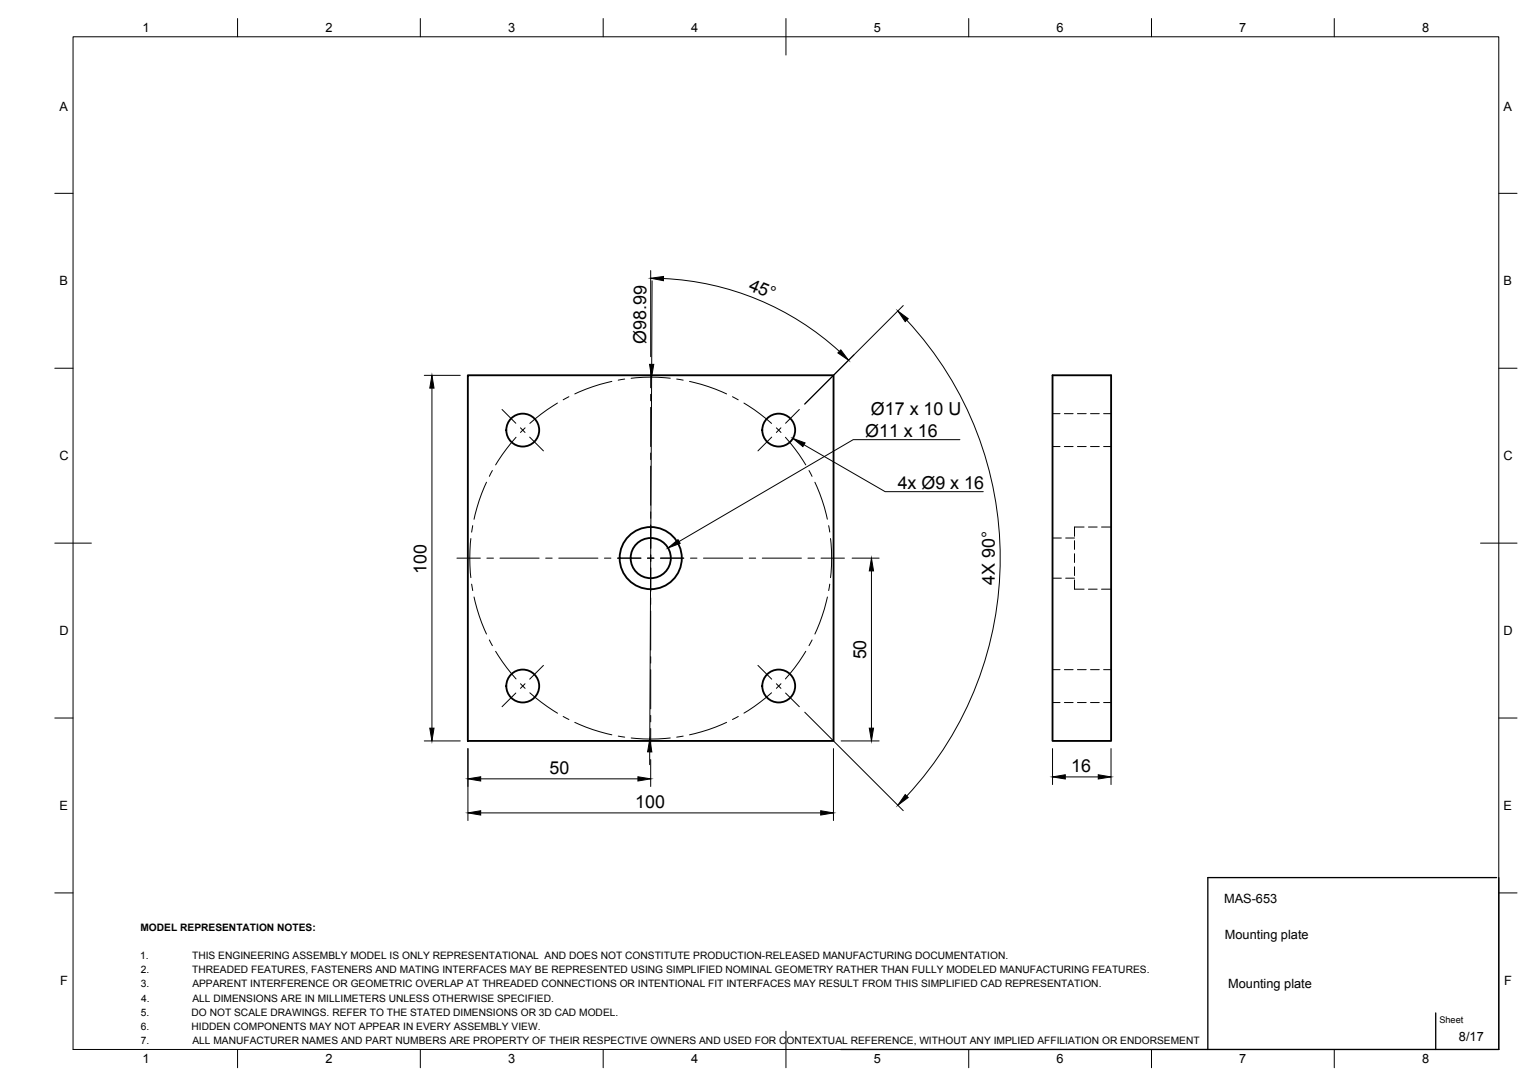
ISO-10303-21;
HEADER;
/* Generated by software containing ST-Developer
 * from STEP Tools, Inc. (www.steptools.com) 
 */

FILE_DESCRIPTION(
/* description */ ('Independent compact industrial fixture table, bolted aluminum worktop
 on connected adjustable support base. Whole-mm nominal dimensions. No
 load rating assigned.'),
/* implementation_level */ '2;1');

FILE_NAME(
/* name */ 'Mounting plate.step',
/* time_stamp */ '2026-11-07T17:47:58-08:00',
/* author */ (''),
/* organization */ (''),
/* preprocessor_version */ 'ST-DEVELOPER v20.2',
/* originating_system */ 'Autodesk Translation Framework v15.17.0.0',
/* authorisation */ '');

FILE_SCHEMA (('AUTOMOTIVE_DESIGN { 1 0 10303 214 3 1 1 }'));
ENDSEC;

DATA;
#10=MECHANICAL_DESIGN_GEOMETRIC_PRESENTATION_REPRESENTATION('',(#2256),#97475);
#2218=SHAPE_REPRESENTATION_RELATIONSHIP('SRR','None',#97612,#2237);
#2237=ADVANCED_BREP_SHAPE_REPRESENTATION('',(#2275),#97462);
#2256=STYLED_ITEM('',(#97722),#2275);
#2275=MANIFOLD_SOLID_BREP('Body1',#21817);
#2328=FACE_BOUND('',#4133,.T.);
#2329=FACE_BOUND('',#4145,.T.);
#2330=FACE_BOUND('',#4146,.T.);
#2331=FACE_BOUND('',#4147,.T.);
#2332=FACE_BOUND('',#4148,.T.);
#2333=FACE_BOUND('',#4149,.T.);
#2334=FACE_BOUND('',#4151,.T.);
#2335=FACE_BOUND('',#4152,.T.);
#2336=FACE_BOUND('',#4153,.T.);
#2337=FACE_BOUND('',#4154,.T.);
#2338=FACE_BOUND('',#4155,.T.);
#2459=PLANE('',#22610);
#2460=PLANE('',#22629);
#2461=PLANE('',#22630);
#2462=PLANE('',#22631);
#2463=PLANE('',#22632);
#2464=PLANE('',#22633);
#2465=PLANE('',#22634);
#2938=FACE_OUTER_BOUND('',#4132,.T.);
#2939=FACE_OUTER_BOUND('',#4134,.T.);
#2940=FACE_OUTER_BOUND('',#4135,.T.);
#2941=FACE_OUTER_BOUND('',#4136,.T.);
#2942=FACE_OUTER_BOUND('',#4137,.T.);
#2943=FACE_OUTER_BOUND('',#4138,.T.);
#2944=FACE_OUTER_BOUND('',#4139,.T.);
#2945=FACE_OUTER_BOUND('',#4140,.T.);
#2946=FACE_OUTER_BOUND('',#4141,.T.);
#2947=FACE_OUTER_BOUND('',#4142,.T.);
#2948=FACE_OUTER_BOUND('',#4143,.T.);
#2949=FACE_OUTER_BOUND('',#4144,.T.);
#2950=FACE_OUTER_BOUND('',#4150,.T.);
#4132=EDGE_LOOP('',(#15422));
#4133=EDGE_LOOP('',(#15423));
#4134=EDGE_LOOP('',(#15424,#15425,#15426,#15427));
#4135=EDGE_LOOP('',(#15428,#15429,#15430,#15431));
#4136=EDGE_LOOP('',(#15432,#15433,#15434,#15435));
#4137=EDGE_LOOP('',(#15436,#15437,#15438,#15439));
#4138=EDGE_LOOP('',(#15440,#15441,#15442,#15443));
#4139=EDGE_LOOP('',(#15444,#15445,#15446,#15447));
#4140=EDGE_LOOP('',(#15448,#15449,#15450,#15451));
#4141=EDGE_LOOP('',(#15452,#15453,#15454,#15455));
#4142=EDGE_LOOP('',(#15456,#15457,#15458,#15459));
#4143=EDGE_LOOP('',(#15460,#15461,#15462,#15463));
#4144=EDGE_LOOP('',(#15464,#15465,#15466,#15467));
#4145=EDGE_LOOP('',(#15468));
#4146=EDGE_LOOP('',(#15469));
#4147=EDGE_LOOP('',(#15470));
#4148=EDGE_LOOP('',(#15471));
#4149=EDGE_LOOP('',(#15472));
#4150=EDGE_LOOP('',(#15473,#15474,#15475,#15476));
#4151=EDGE_LOOP('',(#15477));
#4152=EDGE_LOOP('',(#15478));
#4153=EDGE_LOOP('',(#15479));
#4154=EDGE_LOOP('',(#15480));
#4155=EDGE_LOOP('',(#15481));
#5417=LINE('',#53275,#6631);
#5418=LINE('',#53278,#6632);
#5419=LINE('',#53284,#6633);
#5420=LINE('',#53290,#6634);
#5421=LINE('',#53296,#6635);
#5422=LINE('',#53302,#6636);
#5423=LINE('',#53307,#6637);
#5424=LINE('',#53309,#6638);
#5425=LINE('',#53311,#6639);
#5426=LINE('',#53312,#6640);
#5427=LINE('',#53315,#6641);
#5428=LINE('',#53317,#6642);
#5429=LINE('',#53318,#6643);
#5430=LINE('',#53321,#6644);
#5431=LINE('',#53323,#6645);
#5432=LINE('',#53324,#6646);
#5433=LINE('',#53326,#6647);
#5434=LINE('',#53327,#6648);
#6631=VECTOR('',#25133,8.5);
#6632=VECTOR('',#25136,5.5);
#6633=VECTOR('',#25143,4.5);
#6634=VECTOR('',#25150,4.5);
#6635=VECTOR('',#25157,4.5);
#6636=VECTOR('',#25164,4.5);
#6637=VECTOR('',#25169,10.);
#6638=VECTOR('',#25170,10.);
#6639=VECTOR('',#25171,10.);
#6640=VECTOR('',#25172,10.);
#6641=VECTOR('',#25175,10.);
#6642=VECTOR('',#25176,10.);
#6643=VECTOR('',#25177,10.);
#6644=VECTOR('',#25180,10.);
#6645=VECTOR('',#25181,10.);
#6646=VECTOR('',#25182,10.);
#6647=VECTOR('',#25185,10.);
#6648=VECTOR('',#25186,10.);
#7497=CIRCLE('',#22611,8.5);
#7498=CIRCLE('',#22612,5.5);
#7499=CIRCLE('',#22614,8.5);
#7500=CIRCLE('',#22616,5.5);
#7501=CIRCLE('',#22618,4.5);
#7502=CIRCLE('',#22619,4.5);
#7503=CIRCLE('',#22621,4.5);
#7504=CIRCLE('',#22622,4.5);
#7505=CIRCLE('',#22624,4.5);
#7506=CIRCLE('',#22625,4.5);
#7507=CIRCLE('',#22627,4.5);
#7508=CIRCLE('',#22628,4.5);
#8383=VERTEX_POINT('',#53268);
#8384=VERTEX_POINT('',#53270);
#8385=VERTEX_POINT('',#53273);
#8386=VERTEX_POINT('',#53277);
#8387=VERTEX_POINT('',#53281);
#8388=VERTEX_POINT('',#53283);
#8389=VERTEX_POINT('',#53287);
#8390=VERTEX_POINT('',#53289);
#8391=VERTEX_POINT('',#53293);
#8392=VERTEX_POINT('',#53295);
#8393=VERTEX_POINT('',#53299);
#8394=VERTEX_POINT('',#53301);
#8395=VERTEX_POINT('',#53305);
#8396=VERTEX_POINT('',#53306);
#8397=VERTEX_POINT('',#53308);
#8398=VERTEX_POINT('',#53310);
#8399=VERTEX_POINT('',#53314);
#8400=VERTEX_POINT('',#53316);
#8401=VERTEX_POINT('',#53320);
#8402=VERTEX_POINT('',#53322);
#10968=EDGE_CURVE('',#8383,#8383,#7497,.T.);
#10969=EDGE_CURVE('',#8384,#8384,#7498,.T.);
#10970=EDGE_CURVE('',#8385,#8385,#7499,.T.);
#10971=EDGE_CURVE('',#8385,#8383,#5417,.T.);
#10972=EDGE_CURVE('',#8384,#8386,#5418,.T.);
#10973=EDGE_CURVE('',#8386,#8386,#7500,.T.);
#10974=EDGE_CURVE('',#8387,#8387,#7501,.T.);
#10975=EDGE_CURVE('',#8387,#8388,#5419,.T.);
#10976=EDGE_CURVE('',#8388,#8388,#7502,.T.);
#10977=EDGE_CURVE('',#8389,#8389,#7503,.T.);
#10978=EDGE_CURVE('',#8389,#8390,#5420,.T.);
#10979=EDGE_CURVE('',#8390,#8390,#7504,.T.);
#10980=EDGE_CURVE('',#8391,#8391,#7505,.T.);
#10981=EDGE_CURVE('',#8391,#8392,#5421,.T.);
#10982=EDGE_CURVE('',#8392,#8392,#7506,.T.);
#10983=EDGE_CURVE('',#8393,#8393,#7507,.T.);
#10984=EDGE_CURVE('',#8393,#8394,#5422,.T.);
#10985=EDGE_CURVE('',#8394,#8394,#7508,.T.);
#10986=EDGE_CURVE('',#8395,#8396,#5423,.T.);
#10987=EDGE_CURVE('',#8396,#8397,#5424,.T.);
#10988=EDGE_CURVE('',#8398,#8397,#5425,.T.);
#10989=EDGE_CURVE('',#8395,#8398,#5426,.T.);
#10990=EDGE_CURVE('',#8399,#8395,#5427,.T.);
#10991=EDGE_CURVE('',#8400,#8398,#5428,.T.);
#10992=EDGE_CURVE('',#8399,#8400,#5429,.T.);
#10993=EDGE_CURVE('',#8401,#8399,#5430,.T.);
#10994=EDGE_CURVE('',#8402,#8400,#5431,.T.);
#10995=EDGE_CURVE('',#8401,#8402,#5432,.T.);
#10996=EDGE_CURVE('',#8396,#8401,#5433,.T.);
#10997=EDGE_CURVE('',#8397,#8402,#5434,.T.);
#15422=ORIENTED_EDGE('',*,*,#10968,.F.);
#15423=ORIENTED_EDGE('',*,*,#10969,.T.);
#15424=ORIENTED_EDGE('',*,*,#10970,.F.);
#15425=ORIENTED_EDGE('',*,*,#10971,.T.);
#15426=ORIENTED_EDGE('',*,*,#10968,.T.);
#15427=ORIENTED_EDGE('',*,*,#10971,.F.);
#15428=ORIENTED_EDGE('',*,*,#10969,.F.);
#15429=ORIENTED_EDGE('',*,*,#10972,.T.);
#15430=ORIENTED_EDGE('',*,*,#10973,.F.);
#15431=ORIENTED_EDGE('',*,*,#10972,.F.);
#15432=ORIENTED_EDGE('',*,*,#10974,.F.);
#15433=ORIENTED_EDGE('',*,*,#10975,.T.);
#15434=ORIENTED_EDGE('',*,*,#10976,.F.);
#15435=ORIENTED_EDGE('',*,*,#10975,.F.);
#15436=ORIENTED_EDGE('',*,*,#10977,.F.);
#15437=ORIENTED_EDGE('',*,*,#10978,.T.);
#15438=ORIENTED_EDGE('',*,*,#10979,.F.);
#15439=ORIENTED_EDGE('',*,*,#10978,.F.);
#15440=ORIENTED_EDGE('',*,*,#10980,.F.);
#15441=ORIENTED_EDGE('',*,*,#10981,.T.);
#15442=ORIENTED_EDGE('',*,*,#10982,.F.);
#15443=ORIENTED_EDGE('',*,*,#10981,.F.);
#15444=ORIENTED_EDGE('',*,*,#10983,.F.);
#15445=ORIENTED_EDGE('',*,*,#10984,.T.);
#15446=ORIENTED_EDGE('',*,*,#10985,.F.);
#15447=ORIENTED_EDGE('',*,*,#10984,.F.);
#15448=ORIENTED_EDGE('',*,*,#10986,.T.);
#15449=ORIENTED_EDGE('',*,*,#10987,.T.);
#15450=ORIENTED_EDGE('',*,*,#10988,.F.);
#15451=ORIENTED_EDGE('',*,*,#10989,.F.);
#15452=ORIENTED_EDGE('',*,*,#10990,.T.);
#15453=ORIENTED_EDGE('',*,*,#10989,.T.);
#15454=ORIENTED_EDGE('',*,*,#10991,.F.);
#15455=ORIENTED_EDGE('',*,*,#10992,.F.);
#15456=ORIENTED_EDGE('',*,*,#10993,.T.);
#15457=ORIENTED_EDGE('',*,*,#10992,.T.);
#15458=ORIENTED_EDGE('',*,*,#10994,.F.);
#15459=ORIENTED_EDGE('',*,*,#10995,.F.);
#15460=ORIENTED_EDGE('',*,*,#10996,.T.);
#15461=ORIENTED_EDGE('',*,*,#10995,.T.);
#15462=ORIENTED_EDGE('',*,*,#10997,.F.);
#15463=ORIENTED_EDGE('',*,*,#10987,.F.);
#15464=ORIENTED_EDGE('',*,*,#10997,.T.);
#15465=ORIENTED_EDGE('',*,*,#10994,.T.);
#15466=ORIENTED_EDGE('',*,*,#10991,.T.);
#15467=ORIENTED_EDGE('',*,*,#10988,.T.);
#15468=ORIENTED_EDGE('',*,*,#10970,.T.);
#15469=ORIENTED_EDGE('',*,*,#10974,.T.);
#15470=ORIENTED_EDGE('',*,*,#10977,.T.);
#15471=ORIENTED_EDGE('',*,*,#10980,.T.);
#15472=ORIENTED_EDGE('',*,*,#10983,.T.);
#15473=ORIENTED_EDGE('',*,*,#10996,.F.);
#15474=ORIENTED_EDGE('',*,*,#10986,.F.);
#15475=ORIENTED_EDGE('',*,*,#10990,.F.);
#15476=ORIENTED_EDGE('',*,*,#10993,.F.);
#15477=ORIENTED_EDGE('',*,*,#10973,.T.);
#15478=ORIENTED_EDGE('',*,*,#10976,.T.);
#15479=ORIENTED_EDGE('',*,*,#10979,.T.);
#15480=ORIENTED_EDGE('',*,*,#10982,.T.);
#15481=ORIENTED_EDGE('',*,*,#10985,.T.);
#20016=CYLINDRICAL_SURFACE('',#22613,8.5);
#20017=CYLINDRICAL_SURFACE('',#22615,5.5);
#20018=CYLINDRICAL_SURFACE('',#22617,4.5);
#20019=CYLINDRICAL_SURFACE('',#22620,4.5);
#20020=CYLINDRICAL_SURFACE('',#22623,4.5);
#20021=CYLINDRICAL_SURFACE('',#22626,4.5);
#21058=ADVANCED_FACE('',(#2938,#2328),#2459,.F.);
#21059=ADVANCED_FACE('',(#2939),#20016,.F.);
#21060=ADVANCED_FACE('',(#2940),#20017,.F.);
#21061=ADVANCED_FACE('',(#2941),#20018,.F.);
#21062=ADVANCED_FACE('',(#2942),#20019,.F.);
#21063=ADVANCED_FACE('',(#2943),#20020,.F.);
#21064=ADVANCED_FACE('',(#2944),#20021,.F.);
#21065=ADVANCED_FACE('',(#2945),#2460,.T.);
#21066=ADVANCED_FACE('',(#2946),#2461,.T.);
#21067=ADVANCED_FACE('',(#2947),#2462,.T.);
#21068=ADVANCED_FACE('',(#2948),#2463,.T.);
#21069=ADVANCED_FACE('',(#2949,#2329,#2330,#2331,#2332,#2333),#2464,.T.);
#21070=ADVANCED_FACE('',(#2950,#2334,#2335,#2336,#2337,#2338),#2465,.F.);
#21817=CLOSED_SHELL('',(#21058,#21059,#21060,#21061,#21062,#21063,#21064,
#21065,#21066,#21067,#21068,#21069,#21070));
#22609=AXIS2_PLACEMENT_3D('',#53266,#25121,#25122);
#22610=AXIS2_PLACEMENT_3D('',#53267,#25123,#25124);
#22611=AXIS2_PLACEMENT_3D('',#53269,#25125,#25126);
#22612=AXIS2_PLACEMENT_3D('',#53271,#25127,#25128);
#22613=AXIS2_PLACEMENT_3D('',#53272,#25129,#25130);
#22614=AXIS2_PLACEMENT_3D('',#53274,#25131,#25132);
#22615=AXIS2_PLACEMENT_3D('',#53276,#25134,#25135);
#22616=AXIS2_PLACEMENT_3D('',#53279,#25137,#25138);
#22617=AXIS2_PLACEMENT_3D('',#53280,#25139,#25140);
#22618=AXIS2_PLACEMENT_3D('',#53282,#25141,#25142);
#22619=AXIS2_PLACEMENT_3D('',#53285,#25144,#25145);
#22620=AXIS2_PLACEMENT_3D('',#53286,#25146,#25147);
#22621=AXIS2_PLACEMENT_3D('',#53288,#25148,#25149);
#22622=AXIS2_PLACEMENT_3D('',#53291,#25151,#25152);
#22623=AXIS2_PLACEMENT_3D('',#53292,#25153,#25154);
#22624=AXIS2_PLACEMENT_3D('',#53294,#25155,#25156);
#22625=AXIS2_PLACEMENT_3D('',#53297,#25158,#25159);
#22626=AXIS2_PLACEMENT_3D('',#53298,#25160,#25161);
#22627=AXIS2_PLACEMENT_3D('',#53300,#25162,#25163);
#22628=AXIS2_PLACEMENT_3D('',#53303,#25165,#25166);
#22629=AXIS2_PLACEMENT_3D('',#53304,#25167,#25168);
#22630=AXIS2_PLACEMENT_3D('',#53313,#25173,#25174);
#22631=AXIS2_PLACEMENT_3D('',#53319,#25178,#25179);
#22632=AXIS2_PLACEMENT_3D('',#53325,#25183,#25184);
#22633=AXIS2_PLACEMENT_3D('',#53328,#25187,#25188);
#22634=AXIS2_PLACEMENT_3D('',#53329,#25189,#25190);
#25121=DIRECTION('axis',(0.,0.,1.));
#25122=DIRECTION('refdir',(1.,0.,0.));
#25123=DIRECTION('center_axis',(0.,0.,-1.));
#25124=DIRECTION('ref_axis',(1.,0.,0.));
#25125=DIRECTION('center_axis',(0.,0.,-1.));
#25126=DIRECTION('ref_axis',(1.,0.,0.));
#25127=DIRECTION('center_axis',(0.,0.,-1.));
#25128=DIRECTION('ref_axis',(1.,0.,0.));
#25129=DIRECTION('center_axis',(0.,0.,-1.));
#25130=DIRECTION('ref_axis',(1.,0.,0.));
#25131=DIRECTION('center_axis',(0.,0.,-1.));
#25132=DIRECTION('ref_axis',(1.,0.,0.));
#25133=DIRECTION('',(0.,0.,-1.));
#25134=DIRECTION('center_axis',(0.,0.,-1.));
#25135=DIRECTION('ref_axis',(1.,0.,0.));
#25136=DIRECTION('',(0.,0.,-1.));
#25137=DIRECTION('center_axis',(0.,0.,1.));
#25138=DIRECTION('ref_axis',(1.,0.,0.));
#25139=DIRECTION('center_axis',(0.,0.,-1.));
#25140=DIRECTION('ref_axis',(1.,0.,0.));
#25141=DIRECTION('center_axis',(0.,0.,-1.));
#25142=DIRECTION('ref_axis',(1.,0.,0.));
#25143=DIRECTION('',(0.,0.,-1.));
#25144=DIRECTION('center_axis',(0.,0.,1.));
#25145=DIRECTION('ref_axis',(1.,0.,0.));
#25146=DIRECTION('center_axis',(0.,0.,-1.));
#25147=DIRECTION('ref_axis',(1.,0.,0.));
#25148=DIRECTION('center_axis',(0.,0.,-1.));
#25149=DIRECTION('ref_axis',(1.,0.,0.));
#25150=DIRECTION('',(0.,0.,-1.));
#25151=DIRECTION('center_axis',(0.,0.,1.));
#25152=DIRECTION('ref_axis',(1.,0.,0.));
#25153=DIRECTION('center_axis',(0.,0.,-1.));
#25154=DIRECTION('ref_axis',(1.,0.,0.));
#25155=DIRECTION('center_axis',(0.,0.,-1.));
#25156=DIRECTION('ref_axis',(1.,0.,0.));
#25157=DIRECTION('',(0.,0.,-1.));
#25158=DIRECTION('center_axis',(0.,0.,1.));
#25159=DIRECTION('ref_axis',(1.,0.,0.));
#25160=DIRECTION('center_axis',(0.,0.,-1.));
#25161=DIRECTION('ref_axis',(1.,0.,0.));
#25162=DIRECTION('center_axis',(0.,0.,-1.));
#25163=DIRECTION('ref_axis',(1.,0.,0.));
#25164=DIRECTION('',(0.,0.,-1.));
#25165=DIRECTION('center_axis',(0.,0.,1.));
#25166=DIRECTION('ref_axis',(1.,0.,0.));
#25167=DIRECTION('center_axis',(0.,1.,0.));
#25168=DIRECTION('ref_axis',(-1.,0.,0.));
#25169=DIRECTION('',(-1.,0.,0.));
#25170=DIRECTION('',(0.,0.,1.));
#25171=DIRECTION('',(-1.,0.,0.));
#25172=DIRECTION('',(0.,0.,1.));
#25173=DIRECTION('center_axis',(1.,0.,0.));
#25174=DIRECTION('ref_axis',(0.,1.,0.));
#25175=DIRECTION('',(0.,1.,0.));
#25176=DIRECTION('',(0.,1.,0.));
#25177=DIRECTION('',(0.,0.,1.));
#25178=DIRECTION('center_axis',(0.,-1.,0.));
#25179=DIRECTION('ref_axis',(1.,0.,0.));
#25180=DIRECTION('',(1.,0.,0.));
#25181=DIRECTION('',(1.,0.,0.));
#25182=DIRECTION('',(0.,0.,1.));
#25183=DIRECTION('center_axis',(-1.,0.,0.));
#25184=DIRECTION('ref_axis',(0.,-1.,0.));
#25185=DIRECTION('',(0.,-1.,0.));
#25186=DIRECTION('',(0.,-1.,0.));
#25187=DIRECTION('center_axis',(0.,0.,1.));
#25188=DIRECTION('ref_axis',(1.,0.,0.));
#25189=DIRECTION('center_axis',(0.,0.,1.));
#25190=DIRECTION('ref_axis',(1.,0.,0.));
#53266=CARTESIAN_POINT('',(0.,0.,0.));
#53267=CARTESIAN_POINT('Origin',(0.,0.,6.));
#53268=CARTESIAN_POINT('',(-8.5,1.04094977927525E-15,6.));
#53269=CARTESIAN_POINT('Origin',(0.,0.,6.));
#53270=CARTESIAN_POINT('',(-5.5,6.73555739531044E-16,6.));
#53271=CARTESIAN_POINT('Origin',(0.,0.,6.));
#53272=CARTESIAN_POINT('Origin',(0.,0.,11.));
#53273=CARTESIAN_POINT('',(-8.5,1.04094977927525E-15,16.));
#53274=CARTESIAN_POINT('Origin',(0.,0.,16.));
#53275=CARTESIAN_POINT('',(-8.5,1.04094977927525E-15,11.));
#53276=CARTESIAN_POINT('Origin',(0.,0.,8.));
#53277=CARTESIAN_POINT('',(-5.5,6.73555739531044E-16,0.));
#53278=CARTESIAN_POINT('',(-5.5,6.73555739531044E-16,8.));
#53279=CARTESIAN_POINT('Origin',(0.,0.,0.));
#53280=CARTESIAN_POINT('Origin',(35.,-35.,8.));
#53281=CARTESIAN_POINT('',(30.5,-35.,16.));
#53282=CARTESIAN_POINT('Origin',(35.,-35.,16.));
#53283=CARTESIAN_POINT('',(30.5,-35.,0.));
#53284=CARTESIAN_POINT('',(30.5,-35.,8.));
#53285=CARTESIAN_POINT('Origin',(35.,-35.,0.));
#53286=CARTESIAN_POINT('Origin',(-35.,-35.,8.));
#53287=CARTESIAN_POINT('',(-39.5,-35.,16.));
#53288=CARTESIAN_POINT('Origin',(-35.,-35.,16.));
#53289=CARTESIAN_POINT('',(-39.5,-35.,0.));
#53290=CARTESIAN_POINT('',(-39.5,-35.,8.));
#53291=CARTESIAN_POINT('Origin',(-35.,-35.,0.));
#53292=CARTESIAN_POINT('Origin',(-35.,35.,8.));
#53293=CARTESIAN_POINT('',(-39.5,35.,16.));
#53294=CARTESIAN_POINT('Origin',(-35.,35.,16.));
#53295=CARTESIAN_POINT('',(-39.5,35.,0.));
#53296=CARTESIAN_POINT('',(-39.5,35.,8.));
#53297=CARTESIAN_POINT('Origin',(-35.,35.,0.));
#53298=CARTESIAN_POINT('Origin',(35.,35.,8.));
#53299=CARTESIAN_POINT('',(30.5,35.,16.));
#53300=CARTESIAN_POINT('Origin',(35.,35.,16.));
#53301=CARTESIAN_POINT('',(30.5,35.,0.));
#53302=CARTESIAN_POINT('',(30.5,35.,8.));
#53303=CARTESIAN_POINT('Origin',(35.,35.,0.));
#53304=CARTESIAN_POINT('Origin',(50.,50.,0.));
#53305=CARTESIAN_POINT('',(50.,50.,0.));
#53306=CARTESIAN_POINT('',(-50.,50.,0.));
#53307=CARTESIAN_POINT('',(50.,50.,0.));
#53308=CARTESIAN_POINT('',(-50.,50.,16.));
#53309=CARTESIAN_POINT('',(-50.,50.,0.));
#53310=CARTESIAN_POINT('',(50.,50.,16.));
#53311=CARTESIAN_POINT('',(50.,50.,16.));
#53312=CARTESIAN_POINT('',(50.,50.,0.));
#53313=CARTESIAN_POINT('Origin',(50.,-50.,0.));
#53314=CARTESIAN_POINT('',(50.,-50.,0.));
#53315=CARTESIAN_POINT('',(50.,-50.,0.));
#53316=CARTESIAN_POINT('',(50.,-50.,16.));
#53317=CARTESIAN_POINT('',(50.,-50.,16.));
#53318=CARTESIAN_POINT('',(50.,-50.,0.));
#53319=CARTESIAN_POINT('Origin',(-50.,-50.,0.));
#53320=CARTESIAN_POINT('',(-50.,-50.,0.));
#53321=CARTESIAN_POINT('',(-50.,-50.,0.));
#53322=CARTESIAN_POINT('',(-50.,-50.,16.));
#53323=CARTESIAN_POINT('',(-50.,-50.,16.));
#53324=CARTESIAN_POINT('',(-50.,-50.,0.));
#53325=CARTESIAN_POINT('Origin',(-50.,50.,0.));
#53326=CARTESIAN_POINT('',(-50.,50.,0.));
#53327=CARTESIAN_POINT('',(-50.,50.,16.));
#53328=CARTESIAN_POINT('Origin',(0.,0.,16.));
#53329=CARTESIAN_POINT('Origin',(0.,0.,0.));
#97439=UNCERTAINTY_MEASURE_WITH_UNIT(LENGTH_MEASURE(0.01),#97476,
'DISTANCE_ACCURACY_VALUE',
'Maximum model space distance between geometric entities at asserted c
onnectivities');
#97452=UNCERTAINTY_MEASURE_WITH_UNIT(LENGTH_MEASURE(0.01),#97476,
'DISTANCE_ACCURACY_VALUE',
'Maximum model space distance between geometric entities at asserted c
onnectivities');
#97462=(
GEOMETRIC_REPRESENTATION_CONTEXT(3)
GLOBAL_UNCERTAINTY_ASSIGNED_CONTEXT((#97439))
GLOBAL_UNIT_ASSIGNED_CONTEXT((#97476,#97478,#97479))
REPRESENTATION_CONTEXT('','3D')
);
#97475=(
GEOMETRIC_REPRESENTATION_CONTEXT(3)
GLOBAL_UNCERTAINTY_ASSIGNED_CONTEXT((#97452))
GLOBAL_UNIT_ASSIGNED_CONTEXT((#97476,#97478,#97479))
REPRESENTATION_CONTEXT('','3D')
);
#97476=(
LENGTH_UNIT()
NAMED_UNIT(*)
SI_UNIT(.MILLI.,.METRE.)
);
#97478=(
NAMED_UNIT(*)
PLANE_ANGLE_UNIT()
SI_UNIT($,.RADIAN.)
);
#97479=(
NAMED_UNIT(*)
SI_UNIT($,.STERADIAN.)
SOLID_ANGLE_UNIT()
);
#97489=SHAPE_DEFINITION_REPRESENTATION(#97551,#97612);
#97551=PRODUCT_DEFINITION_SHAPE('',$,#97635);
#97612=SHAPE_REPRESENTATION('',(#22609),#97462);
#97625=PRODUCT_DEFINITION_CONTEXT('part definition',#97693,'design');
#97635=PRODUCT_DEFINITION('Mounting plate','Mounting plate',#97657,#97625);
#97657=PRODUCT_DEFINITION_FORMATION('',$,#97704);
#97693=APPLICATION_CONTEXT(
'Core Data for Automotive Mechanical Design Process');
#97694=PRODUCT_CONTEXT('part definition',#97693,'mechanical');
#97704=PRODUCT('Mounting plate','Mounting plate','Mounting plate',(#97694));
#97722=PRESENTATION_STYLE_ASSIGNMENT((#97729));
#97729=SURFACE_STYLE_USAGE(.BOTH.,#97736);
#97736=SURFACE_SIDE_STYLE('',(#97743));
#97743=SURFACE_STYLE_FILL_AREA(#97750);
#97750=FILL_AREA_STYLE('Gray',(#97757));
#97757=FILL_AREA_STYLE_COLOUR('Gray',#97764);
#97764=COLOUR_RGB('Gray',0.407843137254902,0.447058823529412,0.498039215686275);
ENDSEC;
END-ISO-10303-21;
